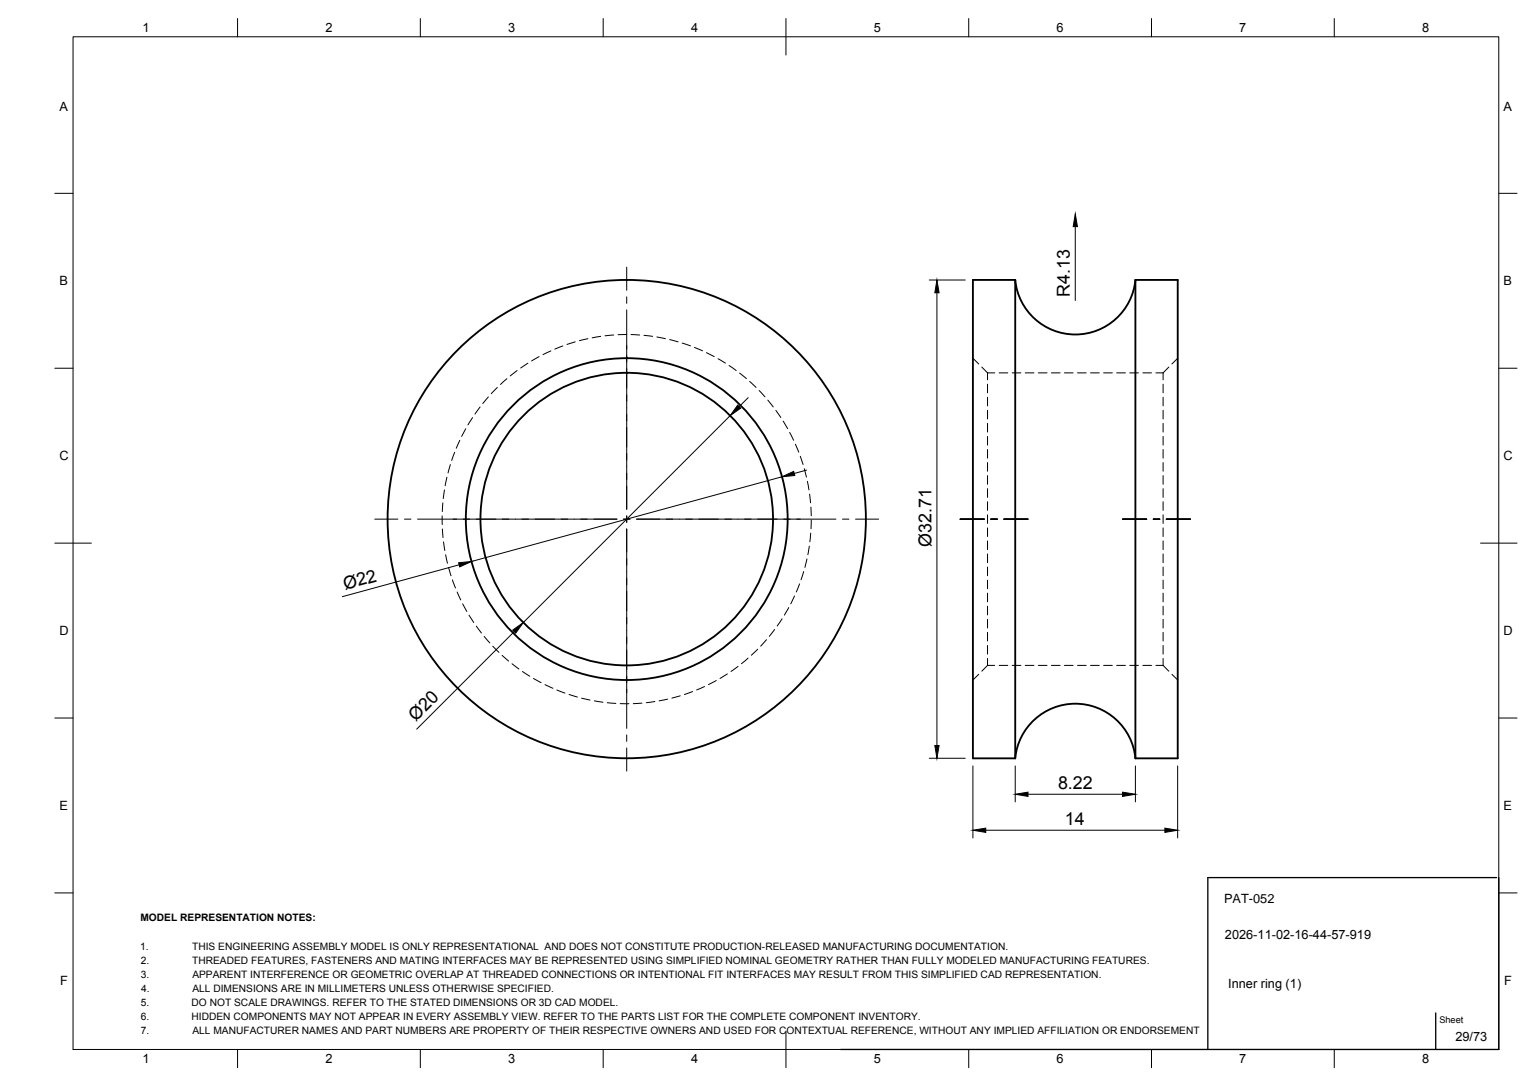
ISO-10303-21;
HEADER;
/* Generated by software containing ST-Developer
 * from STEP Tools, Inc. (www.steptools.com) 
 */

FILE_DESCRIPTION(
/* description */ ('Hand-crank gear train demonstrator'),
/* implementation_level */ '2;1');

FILE_NAME(
/* name */ 'Inner ring (1).step',
/* time_stamp */ '2026-10-28T03:22:13-07:00',
/* author */ (''),
/* organization */ (''),
/* preprocessor_version */ 'ST-DEVELOPER v20.2',
/* originating_system */ 'Autodesk Translation Framework v15.17.0.0',
/* authorisation */ '');

FILE_SCHEMA (('AUTOMOTIVE_DESIGN { 1 0 10303 214 3 1 1 }'));
ENDSEC;

DATA;
#10=MECHANICAL_DESIGN_GEOMETRIC_PRESENTATION_REPRESENTATION('',(#1212),#62758);
#1023=TOROIDAL_SURFACE('',#17614,1.675,0.412776);
#1032=CONICAL_SURFACE('',#17625,1.05,0.785398163397449);
#1033=CONICAL_SURFACE('',#17632,1.05,0.785398163397449);
#1077=SHAPE_REPRESENTATION_RELATIONSHIP('SRR','None',#63051,#1141);
#1141=ADVANCED_BREP_SHAPE_REPRESENTATION('',(#1290),#62705);
#1212=STYLED_ITEM('',(#63462),#1290);
#1290=MANIFOLD_SOLID_BREP('Body1',#16393);
#1496=FACE_BOUND('',#3404,.T.);
#1497=FACE_BOUND('',#3407,.T.);
#1698=PLANE('',#17627);
#1699=PLANE('',#17630);
#2309=FACE_OUTER_BOUND('',#3399,.T.);
#2310=FACE_OUTER_BOUND('',#3400,.T.);
#2311=FACE_OUTER_BOUND('',#3401,.T.);
#2312=FACE_OUTER_BOUND('',#3402,.T.);
#2313=FACE_OUTER_BOUND('',#3403,.T.);
#2314=FACE_OUTER_BOUND('',#3405,.T.);
#2315=FACE_OUTER_BOUND('',#3406,.T.);
#2316=FACE_OUTER_BOUND('',#3408,.T.);
#3399=EDGE_LOOP('',(#11657,#11658,#11659,#11660,#11661,#11662));
#3400=EDGE_LOOP('',(#11663,#11664,#11665,#11666,#11667));
#3401=EDGE_LOOP('',(#11668,#11669,#11670,#11671));
#3402=EDGE_LOOP('',(#11672,#11673,#11674,#11675));
#3403=EDGE_LOOP('',(#11676));
#3404=EDGE_LOOP('',(#11677));
#3405=EDGE_LOOP('',(#11678,#11679,#11680,#11681,#11682));
#3406=EDGE_LOOP('',(#11683));
#3407=EDGE_LOOP('',(#11684));
#3408=EDGE_LOOP('',(#11685,#11686,#11687,#11688));
#4439=LINE('',#24519,#5571);
#4440=LINE('',#24525,#5572);
#4441=LINE('',#24529,#5573);
#4442=LINE('',#24535,#5574);
#4443=LINE('',#24540,#5575);
#5571=VECTOR('',#19910,1.63531);
#5572=VECTOR('',#19917,1.);
#5573=VECTOR('',#19922,1.05);
#5574=VECTOR('',#19931,1.63531);
#5575=VECTOR('',#19938,1.05);
#6794=CIRCLE('',#17615,1.63531);
#6795=CIRCLE('',#17616,1.63531);
#6796=CIRCLE('',#17617,0.412776);
#6797=CIRCLE('',#17618,1.63531);
#6798=CIRCLE('',#17619,1.63531);
#6799=CIRCLE('',#17621,1.63531);
#6800=CIRCLE('',#17623,1.);
#6801=CIRCLE('',#17624,1.);
#6802=CIRCLE('',#17626,1.1);
#6803=CIRCLE('',#17629,1.63531);
#6804=CIRCLE('',#17631,1.1);
#7493=VERTEX_POINT('',#24508);
#7494=VERTEX_POINT('',#24509);
#7495=VERTEX_POINT('',#24512);
#7496=VERTEX_POINT('',#24514);
#7497=VERTEX_POINT('',#24518);
#7498=VERTEX_POINT('',#24522);
#7499=VERTEX_POINT('',#24524);
#7500=VERTEX_POINT('',#24528);
#7501=VERTEX_POINT('',#24533);
#7502=VERTEX_POINT('',#24537);
#9080=EDGE_CURVE('',#7493,#7494,#6794,.T.);
#9081=EDGE_CURVE('',#7494,#7493,#6795,.T.);
#9082=EDGE_CURVE('',#7494,#7495,#6796,.T.);
#9083=EDGE_CURVE('',#7496,#7495,#6797,.T.);
#9084=EDGE_CURVE('',#7495,#7496,#6798,.T.);
#9085=EDGE_CURVE('',#7496,#7497,#4439,.T.);
#9086=EDGE_CURVE('',#7497,#7497,#6799,.T.);
#9087=EDGE_CURVE('',#7498,#7498,#6800,.T.);
#9088=EDGE_CURVE('',#7498,#7499,#4440,.T.);
#9089=EDGE_CURVE('',#7499,#7499,#6801,.T.);
#9090=EDGE_CURVE('',#7499,#7500,#4441,.T.);
#9091=EDGE_CURVE('',#7500,#7500,#6802,.T.);
#9092=EDGE_CURVE('',#7501,#7501,#6803,.T.);
#9093=EDGE_CURVE('',#7501,#7493,#4442,.T.);
#9094=EDGE_CURVE('',#7502,#7502,#6804,.T.);
#9095=EDGE_CURVE('',#7502,#7498,#4443,.T.);
#11657=ORIENTED_EDGE('',*,*,#9080,.F.);
#11658=ORIENTED_EDGE('',*,*,#9081,.F.);
#11659=ORIENTED_EDGE('',*,*,#9082,.T.);
#11660=ORIENTED_EDGE('',*,*,#9083,.F.);
#11661=ORIENTED_EDGE('',*,*,#9084,.F.);
#11662=ORIENTED_EDGE('',*,*,#9082,.F.);
#11663=ORIENTED_EDGE('',*,*,#9083,.T.);
#11664=ORIENTED_EDGE('',*,*,#9084,.T.);
#11665=ORIENTED_EDGE('',*,*,#9085,.T.);
#11666=ORIENTED_EDGE('',*,*,#9086,.T.);
#11667=ORIENTED_EDGE('',*,*,#9085,.F.);
#11668=ORIENTED_EDGE('',*,*,#9087,.T.);
#11669=ORIENTED_EDGE('',*,*,#9088,.T.);
#11670=ORIENTED_EDGE('',*,*,#9089,.F.);
#11671=ORIENTED_EDGE('',*,*,#9088,.F.);
#11672=ORIENTED_EDGE('',*,*,#9089,.T.);
#11673=ORIENTED_EDGE('',*,*,#9090,.T.);
#11674=ORIENTED_EDGE('',*,*,#9091,.F.);
#11675=ORIENTED_EDGE('',*,*,#9090,.F.);
#11676=ORIENTED_EDGE('',*,*,#9086,.F.);
#11677=ORIENTED_EDGE('',*,*,#9091,.T.);
#11678=ORIENTED_EDGE('',*,*,#9092,.F.);
#11679=ORIENTED_EDGE('',*,*,#9093,.T.);
#11680=ORIENTED_EDGE('',*,*,#9080,.T.);
#11681=ORIENTED_EDGE('',*,*,#9081,.T.);
#11682=ORIENTED_EDGE('',*,*,#9093,.F.);
#11683=ORIENTED_EDGE('',*,*,#9092,.T.);
#11684=ORIENTED_EDGE('',*,*,#9094,.F.);
#11685=ORIENTED_EDGE('',*,*,#9094,.T.);
#11686=ORIENTED_EDGE('',*,*,#9095,.T.);
#11687=ORIENTED_EDGE('',*,*,#9087,.F.);
#11688=ORIENTED_EDGE('',*,*,#9095,.F.);
#15265=CYLINDRICAL_SURFACE('',#17620,1.63531);
#15266=CYLINDRICAL_SURFACE('',#17622,1.);
#15267=CYLINDRICAL_SURFACE('',#17628,1.63531);
#15619=ADVANCED_FACE('',(#2309),#1023,.F.);
#15620=ADVANCED_FACE('',(#2310),#15265,.T.);
#15621=ADVANCED_FACE('',(#2311),#15266,.F.);
#15622=ADVANCED_FACE('',(#2312),#1032,.F.);
#15623=ADVANCED_FACE('',(#2313,#1496),#1698,.T.);
#15624=ADVANCED_FACE('',(#2314),#15267,.T.);
#15625=ADVANCED_FACE('',(#2315,#1497),#1699,.T.);
#15626=ADVANCED_FACE('',(#2316),#1033,.F.);
#16393=CLOSED_SHELL('',(#15619,#15620,#15621,#15622,#15623,#15624,#15625,
#15626));
#17613=AXIS2_PLACEMENT_3D('',#24506,#19894,#19895);
#17614=AXIS2_PLACEMENT_3D('',#24507,#19896,#19897);
#17615=AXIS2_PLACEMENT_3D('',#24510,#19898,#19899);
#17616=AXIS2_PLACEMENT_3D('',#24511,#19900,#19901);
#17617=AXIS2_PLACEMENT_3D('',#24513,#19902,#19903);
#17618=AXIS2_PLACEMENT_3D('',#24515,#19904,#19905);
#17619=AXIS2_PLACEMENT_3D('',#24516,#19906,#19907);
#17620=AXIS2_PLACEMENT_3D('',#24517,#19908,#19909);
#17621=AXIS2_PLACEMENT_3D('',#24520,#19911,#19912);
#17622=AXIS2_PLACEMENT_3D('',#24521,#19913,#19914);
#17623=AXIS2_PLACEMENT_3D('',#24523,#19915,#19916);
#17624=AXIS2_PLACEMENT_3D('',#24526,#19918,#19919);
#17625=AXIS2_PLACEMENT_3D('',#24527,#19920,#19921);
#17626=AXIS2_PLACEMENT_3D('',#24530,#19923,#19924);
#17627=AXIS2_PLACEMENT_3D('',#24531,#19925,#19926);
#17628=AXIS2_PLACEMENT_3D('',#24532,#19927,#19928);
#17629=AXIS2_PLACEMENT_3D('',#24534,#19929,#19930);
#17630=AXIS2_PLACEMENT_3D('',#24536,#19932,#19933);
#17631=AXIS2_PLACEMENT_3D('',#24538,#19934,#19935);
#17632=AXIS2_PLACEMENT_3D('',#24539,#19936,#19937);
#19894=DIRECTION('axis',(0.,0.,1.));
#19895=DIRECTION('refdir',(1.,0.,0.));
#19896=DIRECTION('center_axis',(0.,-1.,0.));
#19897=DIRECTION('ref_axis',(0.,0.,-1.));
#19898=DIRECTION('center_axis',(0.,-1.,0.));
#19899=DIRECTION('ref_axis',(1.,0.,0.));
#19900=DIRECTION('center_axis',(0.,-1.,0.));
#19901=DIRECTION('ref_axis',(1.,0.,0.));
#19902=DIRECTION('center_axis',(1.,0.,1.22464679914735E-16));
#19903=DIRECTION('ref_axis',(-1.22464679914735E-16,0.,1.));
#19904=DIRECTION('center_axis',(0.,1.,0.));
#19905=DIRECTION('ref_axis',(1.,0.,0.));
#19906=DIRECTION('center_axis',(0.,1.,0.));
#19907=DIRECTION('ref_axis',(1.,0.,0.));
#19908=DIRECTION('center_axis',(0.,-1.,0.));
#19909=DIRECTION('ref_axis',(1.,0.,0.));
#19910=DIRECTION('',(0.,1.,0.));
#19911=DIRECTION('center_axis',(0.,-1.,0.));
#19912=DIRECTION('ref_axis',(1.,0.,0.));
#19913=DIRECTION('center_axis',(0.,-1.,0.));
#19914=DIRECTION('ref_axis',(1.,0.,0.));
#19915=DIRECTION('center_axis',(0.,-1.,0.));
#19916=DIRECTION('ref_axis',(1.,0.,0.));
#19917=DIRECTION('',(0.,1.,0.));
#19918=DIRECTION('center_axis',(0.,-1.,0.));
#19919=DIRECTION('ref_axis',(1.,0.,0.));
#19920=DIRECTION('center_axis',(0.,1.,0.));
#19921=DIRECTION('ref_axis',(1.,0.,0.));
#19922=DIRECTION('',(-0.707106781186548,0.707106781186547,-8.65956056235494E-17));
#19923=DIRECTION('center_axis',(0.,-1.,0.));
#19924=DIRECTION('ref_axis',(1.,0.,0.));
#19925=DIRECTION('center_axis',(0.,1.,0.));
#19926=DIRECTION('ref_axis',(0.,0.,1.));
#19927=DIRECTION('center_axis',(0.,-1.,0.));
#19928=DIRECTION('ref_axis',(1.,0.,0.));
#19929=DIRECTION('center_axis',(0.,-1.,0.));
#19930=DIRECTION('ref_axis',(1.,0.,0.));
#19931=DIRECTION('',(0.,1.,0.));
#19932=DIRECTION('center_axis',(0.,-1.,0.));
#19933=DIRECTION('ref_axis',(0.,0.,-1.));
#19934=DIRECTION('center_axis',(0.,-1.,0.));
#19935=DIRECTION('ref_axis',(1.,0.,0.));
#19936=DIRECTION('center_axis',(0.,-1.,0.));
#19937=DIRECTION('ref_axis',(1.,0.,0.));
#19938=DIRECTION('',(0.707106781186548,0.707106781186547,8.65956056235494E-17));
#24506=CARTESIAN_POINT('',(0.,0.,0.));
#24507=CARTESIAN_POINT('Origin',(0.,0.,0.));
#24508=CARTESIAN_POINT('',(-1.63531,-0.410863395882378,-2.00267715711366E-16));
#24509=CARTESIAN_POINT('',(-2.00267715711366E-16,-0.410863395882378,1.63531));
#24510=CARTESIAN_POINT('Origin',(0.,-0.410863395882378,0.));
#24511=CARTESIAN_POINT('Origin',(0.,-0.410863395882378,0.));
#24512=CARTESIAN_POINT('',(-2.00267715711366E-16,0.410863395882378,1.63531));
#24513=CARTESIAN_POINT('Origin',(-2.05128338857182E-16,0.,1.675));
#24514=CARTESIAN_POINT('',(-1.63531,0.410863395882378,2.00267715711366E-16));
#24515=CARTESIAN_POINT('Origin',(0.,0.410863395882378,0.));
#24516=CARTESIAN_POINT('Origin',(0.,0.410863395882378,0.));
#24517=CARTESIAN_POINT('Origin',(0.,0.,0.));
#24518=CARTESIAN_POINT('',(-1.63531,0.7,-2.00267715711366E-16));
#24519=CARTESIAN_POINT('',(-1.63531,0.,-2.00267715711366E-16));
#24520=CARTESIAN_POINT('Origin',(0.,0.7,0.));
#24521=CARTESIAN_POINT('Origin',(0.,0.,0.));
#24522=CARTESIAN_POINT('',(-1.,-0.6,-1.22464679914735E-16));
#24523=CARTESIAN_POINT('Origin',(0.,-0.6,0.));
#24524=CARTESIAN_POINT('',(-1.,0.6,-1.22464679914735E-16));
#24525=CARTESIAN_POINT('',(-1.,0.,-1.22464679914735E-16));
#24526=CARTESIAN_POINT('Origin',(0.,0.6,0.));
#24527=CARTESIAN_POINT('Origin',(0.,0.65,0.));
#24528=CARTESIAN_POINT('',(-1.1,0.7,-1.34711147906209E-16));
#24529=CARTESIAN_POINT('',(-1.05,0.65,-1.28587913910472E-16));
#24530=CARTESIAN_POINT('Origin',(0.,0.7,0.));
#24531=CARTESIAN_POINT('Origin',(1.63531,0.7,0.));
#24532=CARTESIAN_POINT('Origin',(0.,0.,0.));
#24533=CARTESIAN_POINT('',(-1.63531,-0.7,-2.00267715711366E-16));
#24534=CARTESIAN_POINT('Origin',(0.,-0.7,0.));
#24535=CARTESIAN_POINT('',(-1.63531,0.,-2.00267715711366E-16));
#24536=CARTESIAN_POINT('Origin',(1.1,-0.7,0.));
#24537=CARTESIAN_POINT('',(-1.1,-0.7,-1.34711147906209E-16));
#24538=CARTESIAN_POINT('Origin',(0.,-0.7,0.));
#24539=CARTESIAN_POINT('Origin',(0.,-0.65,0.));
#24540=CARTESIAN_POINT('',(-1.05,-0.65,-1.28587913910472E-16));
#62631=UNCERTAINTY_MEASURE_WITH_UNIT(LENGTH_MEASURE(0.001),#62759,
'DISTANCE_ACCURACY_VALUE',
'Maximum model space distance between geometric entities at asserted c
onnectivities');
#62684=UNCERTAINTY_MEASURE_WITH_UNIT(LENGTH_MEASURE(0.001),#62759,
'DISTANCE_ACCURACY_VALUE',
'Maximum model space distance between geometric entities at asserted c
onnectivities');
#62705=(
GEOMETRIC_REPRESENTATION_CONTEXT(3)
GLOBAL_UNCERTAINTY_ASSIGNED_CONTEXT((#62631))
GLOBAL_UNIT_ASSIGNED_CONTEXT((#62759,#62761,#62762))
REPRESENTATION_CONTEXT('','3D')
);
#62758=(
GEOMETRIC_REPRESENTATION_CONTEXT(3)
GLOBAL_UNCERTAINTY_ASSIGNED_CONTEXT((#62684))
GLOBAL_UNIT_ASSIGNED_CONTEXT((#62759,#62761,#62762))
REPRESENTATION_CONTEXT('','3D')
);
#62759=(
LENGTH_UNIT()
NAMED_UNIT(*)
SI_UNIT(.CENTI.,.METRE.)
);
#62761=(
NAMED_UNIT(*)
PLANE_ANGLE_UNIT()
SI_UNIT($,.RADIAN.)
);
#62762=(
NAMED_UNIT(*)
SI_UNIT($,.STERADIAN.)
SOLID_ANGLE_UNIT()
);
#62783=SHAPE_DEFINITION_REPRESENTATION(#62861,#63051);
#62861=PRODUCT_DEFINITION_SHAPE('',$,#63125);
#63051=SHAPE_REPRESENTATION('',(#17613),#62705);
#63104=PRODUCT_DEFINITION_CONTEXT('part definition',#63325,'design');
#63125=PRODUCT_DEFINITION('Inner ring (1)','Inner ring (1)',#63198,#63104);
#63198=PRODUCT_DEFINITION_FORMATION('',$,#63347);
#63325=APPLICATION_CONTEXT(
'Core Data for Automotive Mechanical Design Process');
#63326=PRODUCT_CONTEXT('part definition',#63325,'mechanical');
#63347=PRODUCT('Inner ring (1)','Inner ring (1)','Inner ring (1)',(#63326));
#63456=COLOUR_RGB('Grey',0.48,0.52,0.57);
#63457=FILL_AREA_STYLE_COLOUR('',#63456);
#63458=FILL_AREA_STYLE('',(#63457));
#63459=SURFACE_STYLE_FILL_AREA(#63458);
#63460=SURFACE_SIDE_STYLE('',(#63459));
#63461=SURFACE_STYLE_USAGE(.BOTH.,#63460);
#63462=PRESENTATION_STYLE_ASSIGNMENT((#63461));
ENDSEC;
END-ISO-10303-21;
